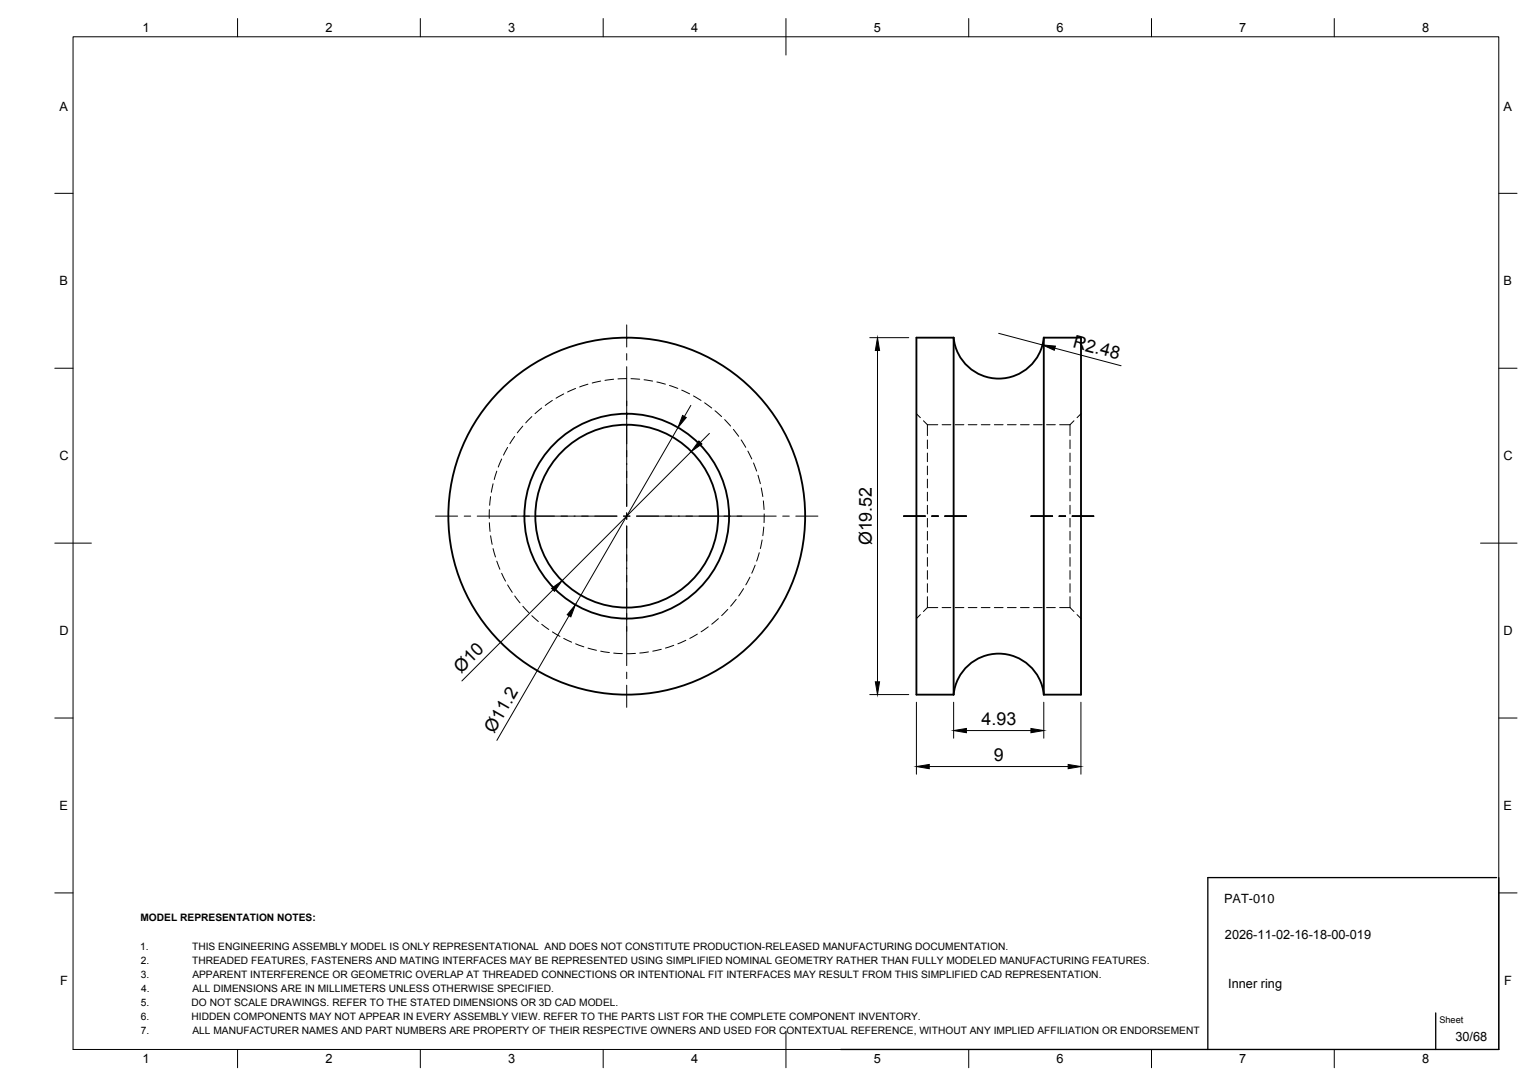
ISO-10303-21;
HEADER;
/* Generated by software containing ST-Developer
 * from STEP Tools, Inc. (www.steptools.com) 
 */

FILE_DESCRIPTION(
/* description */ ('Belt conveyor head drive unit'),
/* implementation_level */ '2;1');

FILE_NAME(
/* name */ 'Inner ring.step',
/* time_stamp */ '2026-10-28T03:26:19-07:00',
/* author */ (''),
/* organization */ (''),
/* preprocessor_version */ 'ST-DEVELOPER v20.2',
/* originating_system */ 'Autodesk Translation Framework v15.17.0.0',
/* authorisation */ '');

FILE_SCHEMA (('AUTOMOTIVE_DESIGN { 1 0 10303 214 3 1 1 }'));
ENDSEC;

DATA;
#10=MECHANICAL_DESIGN_GEOMETRIC_PRESENTATION_REPRESENTATION('',(#874),#27069);
#677=CONICAL_SURFACE('',#15202,0.53,0.785398163397448);
#678=CONICAL_SURFACE('',#15209,0.53,0.785398163397448);
#705=TOROIDAL_SURFACE('',#15191,1.,0.247676);
#736=SHAPE_REPRESENTATION_RELATIONSHIP('SRR','None',#27381,#805);
#805=ADVANCED_BREP_SHAPE_REPRESENTATION('',(#959),#27023);
#874=STYLED_ITEM('',(#27797),#959);
#959=MANIFOLD_SOLID_BREP('Body1',#13739);
#1151=FACE_BOUND('',#2879,.T.);
#1152=FACE_BOUND('',#2882,.T.);
#1437=PLANE('',#15204);
#1438=PLANE('',#15207);
#1935=FACE_OUTER_BOUND('',#2874,.T.);
#1936=FACE_OUTER_BOUND('',#2875,.T.);
#1937=FACE_OUTER_BOUND('',#2876,.T.);
#1938=FACE_OUTER_BOUND('',#2877,.T.);
#1939=FACE_OUTER_BOUND('',#2878,.T.);
#1940=FACE_OUTER_BOUND('',#2880,.T.);
#1941=FACE_OUTER_BOUND('',#2881,.T.);
#1942=FACE_OUTER_BOUND('',#2883,.T.);
#2874=EDGE_LOOP('',(#10272,#10273,#10274,#10275,#10276,#10277));
#2875=EDGE_LOOP('',(#10278,#10279,#10280,#10281,#10282));
#2876=EDGE_LOOP('',(#10283,#10284,#10285,#10286));
#2877=EDGE_LOOP('',(#10287,#10288,#10289,#10290));
#2878=EDGE_LOOP('',(#10291));
#2879=EDGE_LOOP('',(#10292));
#2880=EDGE_LOOP('',(#10293,#10294,#10295,#10296,#10297));
#2881=EDGE_LOOP('',(#10298));
#2882=EDGE_LOOP('',(#10299));
#2883=EDGE_LOOP('',(#10300,#10301,#10302,#10303));
#3859=LINE('',#22410,#4651);
#3860=LINE('',#22416,#4652);
#3861=LINE('',#22420,#4653);
#3862=LINE('',#22426,#4654);
#3863=LINE('',#22431,#4655);
#4651=VECTOR('',#18067,0.976185);
#4652=VECTOR('',#18074,0.5);
#4653=VECTOR('',#18079,0.53);
#4654=VECTOR('',#18088,0.976185);
#4655=VECTOR('',#18095,0.53);
#5378=CIRCLE('',#15192,0.976185);
#5379=CIRCLE('',#15193,0.976185);
#5380=CIRCLE('',#15194,0.247676);
#5381=CIRCLE('',#15195,0.976185);
#5382=CIRCLE('',#15196,0.976185);
#5383=CIRCLE('',#15198,0.976185);
#5384=CIRCLE('',#15200,0.5);
#5385=CIRCLE('',#15201,0.5);
#5386=CIRCLE('',#15203,0.56);
#5387=CIRCLE('',#15206,0.976185);
#5388=CIRCLE('',#15208,0.56);
#6391=VERTEX_POINT('',#22399);
#6392=VERTEX_POINT('',#22400);
#6393=VERTEX_POINT('',#22403);
#6394=VERTEX_POINT('',#22405);
#6395=VERTEX_POINT('',#22409);
#6396=VERTEX_POINT('',#22413);
#6397=VERTEX_POINT('',#22415);
#6398=VERTEX_POINT('',#22419);
#6399=VERTEX_POINT('',#22424);
#6400=VERTEX_POINT('',#22428);
#7828=EDGE_CURVE('',#6391,#6392,#5378,.T.);
#7829=EDGE_CURVE('',#6392,#6391,#5379,.T.);
#7830=EDGE_CURVE('',#6392,#6393,#5380,.T.);
#7831=EDGE_CURVE('',#6394,#6393,#5381,.T.);
#7832=EDGE_CURVE('',#6393,#6394,#5382,.T.);
#7833=EDGE_CURVE('',#6394,#6395,#3859,.T.);
#7834=EDGE_CURVE('',#6395,#6395,#5383,.T.);
#7835=EDGE_CURVE('',#6396,#6396,#5384,.T.);
#7836=EDGE_CURVE('',#6396,#6397,#3860,.T.);
#7837=EDGE_CURVE('',#6397,#6397,#5385,.T.);
#7838=EDGE_CURVE('',#6397,#6398,#3861,.T.);
#7839=EDGE_CURVE('',#6398,#6398,#5386,.T.);
#7840=EDGE_CURVE('',#6399,#6399,#5387,.T.);
#7841=EDGE_CURVE('',#6399,#6391,#3862,.T.);
#7842=EDGE_CURVE('',#6400,#6400,#5388,.T.);
#7843=EDGE_CURVE('',#6400,#6396,#3863,.T.);
#10272=ORIENTED_EDGE('',*,*,#7828,.F.);
#10273=ORIENTED_EDGE('',*,*,#7829,.F.);
#10274=ORIENTED_EDGE('',*,*,#7830,.T.);
#10275=ORIENTED_EDGE('',*,*,#7831,.F.);
#10276=ORIENTED_EDGE('',*,*,#7832,.F.);
#10277=ORIENTED_EDGE('',*,*,#7830,.F.);
#10278=ORIENTED_EDGE('',*,*,#7831,.T.);
#10279=ORIENTED_EDGE('',*,*,#7832,.T.);
#10280=ORIENTED_EDGE('',*,*,#7833,.T.);
#10281=ORIENTED_EDGE('',*,*,#7834,.T.);
#10282=ORIENTED_EDGE('',*,*,#7833,.F.);
#10283=ORIENTED_EDGE('',*,*,#7835,.T.);
#10284=ORIENTED_EDGE('',*,*,#7836,.T.);
#10285=ORIENTED_EDGE('',*,*,#7837,.F.);
#10286=ORIENTED_EDGE('',*,*,#7836,.F.);
#10287=ORIENTED_EDGE('',*,*,#7837,.T.);
#10288=ORIENTED_EDGE('',*,*,#7838,.T.);
#10289=ORIENTED_EDGE('',*,*,#7839,.F.);
#10290=ORIENTED_EDGE('',*,*,#7838,.F.);
#10291=ORIENTED_EDGE('',*,*,#7834,.F.);
#10292=ORIENTED_EDGE('',*,*,#7839,.T.);
#10293=ORIENTED_EDGE('',*,*,#7840,.F.);
#10294=ORIENTED_EDGE('',*,*,#7841,.T.);
#10295=ORIENTED_EDGE('',*,*,#7828,.T.);
#10296=ORIENTED_EDGE('',*,*,#7829,.T.);
#10297=ORIENTED_EDGE('',*,*,#7841,.F.);
#10298=ORIENTED_EDGE('',*,*,#7840,.T.);
#10299=ORIENTED_EDGE('',*,*,#7842,.F.);
#10300=ORIENTED_EDGE('',*,*,#7842,.T.);
#10301=ORIENTED_EDGE('',*,*,#7843,.T.);
#10302=ORIENTED_EDGE('',*,*,#7835,.F.);
#10303=ORIENTED_EDGE('',*,*,#7843,.F.);
#12674=CYLINDRICAL_SURFACE('',#15197,0.976185);
#12675=CYLINDRICAL_SURFACE('',#15199,0.5);
#12676=CYLINDRICAL_SURFACE('',#15205,0.976185);
#13214=ADVANCED_FACE('',(#1935),#705,.F.);
#13215=ADVANCED_FACE('',(#1936),#12674,.T.);
#13216=ADVANCED_FACE('',(#1937),#12675,.F.);
#13217=ADVANCED_FACE('',(#1938),#677,.F.);
#13218=ADVANCED_FACE('',(#1939,#1151),#1437,.T.);
#13219=ADVANCED_FACE('',(#1940),#12676,.T.);
#13220=ADVANCED_FACE('',(#1941,#1152),#1438,.T.);
#13221=ADVANCED_FACE('',(#1942),#678,.F.);
#13739=CLOSED_SHELL('',(#13214,#13215,#13216,#13217,#13218,#13219,#13220,
#13221));
#15190=AXIS2_PLACEMENT_3D('',#22397,#18051,#18052);
#15191=AXIS2_PLACEMENT_3D('',#22398,#18053,#18054);
#15192=AXIS2_PLACEMENT_3D('',#22401,#18055,#18056);
#15193=AXIS2_PLACEMENT_3D('',#22402,#18057,#18058);
#15194=AXIS2_PLACEMENT_3D('',#22404,#18059,#18060);
#15195=AXIS2_PLACEMENT_3D('',#22406,#18061,#18062);
#15196=AXIS2_PLACEMENT_3D('',#22407,#18063,#18064);
#15197=AXIS2_PLACEMENT_3D('',#22408,#18065,#18066);
#15198=AXIS2_PLACEMENT_3D('',#22411,#18068,#18069);
#15199=AXIS2_PLACEMENT_3D('',#22412,#18070,#18071);
#15200=AXIS2_PLACEMENT_3D('',#22414,#18072,#18073);
#15201=AXIS2_PLACEMENT_3D('',#22417,#18075,#18076);
#15202=AXIS2_PLACEMENT_3D('',#22418,#18077,#18078);
#15203=AXIS2_PLACEMENT_3D('',#22421,#18080,#18081);
#15204=AXIS2_PLACEMENT_3D('',#22422,#18082,#18083);
#15205=AXIS2_PLACEMENT_3D('',#22423,#18084,#18085);
#15206=AXIS2_PLACEMENT_3D('',#22425,#18086,#18087);
#15207=AXIS2_PLACEMENT_3D('',#22427,#18089,#18090);
#15208=AXIS2_PLACEMENT_3D('',#22429,#18091,#18092);
#15209=AXIS2_PLACEMENT_3D('',#22430,#18093,#18094);
#18051=DIRECTION('axis',(0.,0.,1.));
#18052=DIRECTION('refdir',(1.,0.,0.));
#18053=DIRECTION('center_axis',(0.,-1.,0.));
#18054=DIRECTION('ref_axis',(0.,0.,-1.));
#18055=DIRECTION('center_axis',(0.,-1.,0.));
#18056=DIRECTION('ref_axis',(1.,0.,0.));
#18057=DIRECTION('center_axis',(0.,-1.,0.));
#18058=DIRECTION('ref_axis',(1.,0.,0.));
#18059=DIRECTION('center_axis',(1.,0.,1.22464679914735E-16));
#18060=DIRECTION('ref_axis',(-1.22464679914735E-16,0.,1.));
#18061=DIRECTION('center_axis',(0.,1.,0.));
#18062=DIRECTION('ref_axis',(1.,0.,0.));
#18063=DIRECTION('center_axis',(0.,1.,0.));
#18064=DIRECTION('ref_axis',(1.,0.,0.));
#18065=DIRECTION('center_axis',(0.,-1.,0.));
#18066=DIRECTION('ref_axis',(1.,0.,0.));
#18067=DIRECTION('',(0.,1.,0.));
#18068=DIRECTION('center_axis',(0.,-1.,0.));
#18069=DIRECTION('ref_axis',(1.,0.,0.));
#18070=DIRECTION('center_axis',(0.,-1.,0.));
#18071=DIRECTION('ref_axis',(1.,0.,0.));
#18072=DIRECTION('center_axis',(0.,-1.,0.));
#18073=DIRECTION('ref_axis',(1.,0.,0.));
#18074=DIRECTION('',(0.,1.,0.));
#18075=DIRECTION('center_axis',(0.,-1.,0.));
#18076=DIRECTION('ref_axis',(1.,0.,0.));
#18077=DIRECTION('center_axis',(0.,1.,0.));
#18078=DIRECTION('ref_axis',(1.,0.,0.));
#18079=DIRECTION('',(-0.707106781186547,0.707106781186548,-8.65956056235493E-17));
#18080=DIRECTION('center_axis',(0.,-1.,0.));
#18081=DIRECTION('ref_axis',(1.,0.,0.));
#18082=DIRECTION('center_axis',(0.,1.,0.));
#18083=DIRECTION('ref_axis',(0.,0.,1.));
#18084=DIRECTION('center_axis',(0.,-1.,0.));
#18085=DIRECTION('ref_axis',(1.,0.,0.));
#18086=DIRECTION('center_axis',(0.,-1.,0.));
#18087=DIRECTION('ref_axis',(1.,0.,0.));
#18088=DIRECTION('',(0.,1.,0.));
#18089=DIRECTION('center_axis',(0.,-1.,0.));
#18090=DIRECTION('ref_axis',(0.,0.,-1.));
#18091=DIRECTION('center_axis',(0.,-1.,0.));
#18092=DIRECTION('ref_axis',(1.,0.,0.));
#18093=DIRECTION('center_axis',(0.,-1.,0.));
#18094=DIRECTION('ref_axis',(1.,0.,0.));
#18095=DIRECTION('',(0.707106781186547,0.707106781186548,8.65956056235493E-17));
#22397=CARTESIAN_POINT('',(0.,0.,0.));
#22398=CARTESIAN_POINT('Origin',(0.,0.,0.));
#22399=CARTESIAN_POINT('',(-0.976185,-0.246528389340863,-1.19548183562566E-16));
#22400=CARTESIAN_POINT('',(-1.19548183562566E-16,-0.246528389340863,0.976185));
#22401=CARTESIAN_POINT('Origin',(0.,-0.246528389340863,0.));
#22402=CARTESIAN_POINT('Origin',(0.,-0.246528389340863,0.));
#22403=CARTESIAN_POINT('',(-1.19548183562566E-16,0.246528389340863,0.976185));
#22404=CARTESIAN_POINT('Origin',(-1.22464679914735E-16,0.,1.));
#22405=CARTESIAN_POINT('',(-0.976185,0.246528389340863,1.19548183562566E-16));
#22406=CARTESIAN_POINT('Origin',(0.,0.246528389340863,0.));
#22407=CARTESIAN_POINT('Origin',(0.,0.246528389340863,0.));
#22408=CARTESIAN_POINT('Origin',(0.,0.,0.));
#22409=CARTESIAN_POINT('',(-0.976185,0.45,-1.19548183562566E-16));
#22410=CARTESIAN_POINT('',(-0.976185,0.,-1.19548183562566E-16));
#22411=CARTESIAN_POINT('Origin',(0.,0.45,0.));
#22412=CARTESIAN_POINT('Origin',(0.,0.,0.));
#22413=CARTESIAN_POINT('',(-0.5,-0.39,-6.12323399573677E-17));
#22414=CARTESIAN_POINT('Origin',(0.,-0.39,0.));
#22415=CARTESIAN_POINT('',(-0.5,0.39,-6.12323399573677E-17));
#22416=CARTESIAN_POINT('',(-0.5,0.,-6.12323399573677E-17));
#22417=CARTESIAN_POINT('Origin',(0.,0.39,0.));
#22418=CARTESIAN_POINT('Origin',(0.,0.42,0.));
#22419=CARTESIAN_POINT('',(-0.56,0.45,-6.85802207522518E-17));
#22420=CARTESIAN_POINT('',(-0.53,0.42,-6.49062803548097E-17));
#22421=CARTESIAN_POINT('Origin',(0.,0.45,0.));
#22422=CARTESIAN_POINT('Origin',(0.976185,0.45,0.));
#22423=CARTESIAN_POINT('Origin',(0.,0.,0.));
#22424=CARTESIAN_POINT('',(-0.976185,-0.45,-1.19548183562566E-16));
#22425=CARTESIAN_POINT('Origin',(0.,-0.45,0.));
#22426=CARTESIAN_POINT('',(-0.976185,0.,-1.19548183562566E-16));
#22427=CARTESIAN_POINT('Origin',(0.56,-0.45,0.));
#22428=CARTESIAN_POINT('',(-0.56,-0.45,-6.85802207522518E-17));
#22429=CARTESIAN_POINT('Origin',(0.,-0.45,0.));
#22430=CARTESIAN_POINT('Origin',(0.,-0.42,0.));
#22431=CARTESIAN_POINT('',(-0.53,-0.42,-6.49062803548097E-17));
#26946=UNCERTAINTY_MEASURE_WITH_UNIT(LENGTH_MEASURE(0.001),#27070,
'DISTANCE_ACCURACY_VALUE',
'Maximum model space distance between geometric entities at asserted c
onnectivities');
#26992=UNCERTAINTY_MEASURE_WITH_UNIT(LENGTH_MEASURE(0.001),#27070,
'DISTANCE_ACCURACY_VALUE',
'Maximum model space distance between geometric entities at asserted c
onnectivities');
#27023=(
GEOMETRIC_REPRESENTATION_CONTEXT(3)
GLOBAL_UNCERTAINTY_ASSIGNED_CONTEXT((#26946))
GLOBAL_UNIT_ASSIGNED_CONTEXT((#27070,#27072,#27073))
REPRESENTATION_CONTEXT('','3D')
);
#27069=(
GEOMETRIC_REPRESENTATION_CONTEXT(3)
GLOBAL_UNCERTAINTY_ASSIGNED_CONTEXT((#26992))
GLOBAL_UNIT_ASSIGNED_CONTEXT((#27070,#27072,#27073))
REPRESENTATION_CONTEXT('','3D')
);
#27070=(
LENGTH_UNIT()
NAMED_UNIT(*)
SI_UNIT(.CENTI.,.METRE.)
);
#27072=(
NAMED_UNIT(*)
PLANE_ANGLE_UNIT()
SI_UNIT($,.RADIAN.)
);
#27073=(
NAMED_UNIT(*)
SI_UNIT($,.STERADIAN.)
SOLID_ANGLE_UNIT()
);
#27104=SHAPE_DEFINITION_REPRESENTATION(#27180,#27381);
#27180=PRODUCT_DEFINITION_SHAPE('',$,#27458);
#27381=SHAPE_REPRESENTATION('',(#15190),#27023);
#27427=PRODUCT_DEFINITION_CONTEXT('part definition',#27657,'design');
#27458=PRODUCT_DEFINITION('Inner ring','Inner ring',#27534,#27427);
#27534=PRODUCT_DEFINITION_FORMATION('',$,#27689);
#27657=APPLICATION_CONTEXT(
'Core Data for Automotive Mechanical Design Process');
#27658=PRODUCT_CONTEXT('part definition',#27657,'mechanical');
#27689=PRODUCT('Inner ring','Inner ring','Inner ring',(#27658));
#27791=COLOUR_RGB('Grey',0.48,0.52,0.57);
#27792=FILL_AREA_STYLE_COLOUR('',#27791);
#27793=FILL_AREA_STYLE('',(#27792));
#27794=SURFACE_STYLE_FILL_AREA(#27793);
#27795=SURFACE_SIDE_STYLE('',(#27794));
#27796=SURFACE_STYLE_USAGE(.BOTH.,#27795);
#27797=PRESENTATION_STYLE_ASSIGNMENT((#27796));
ENDSEC;
END-ISO-10303-21;
